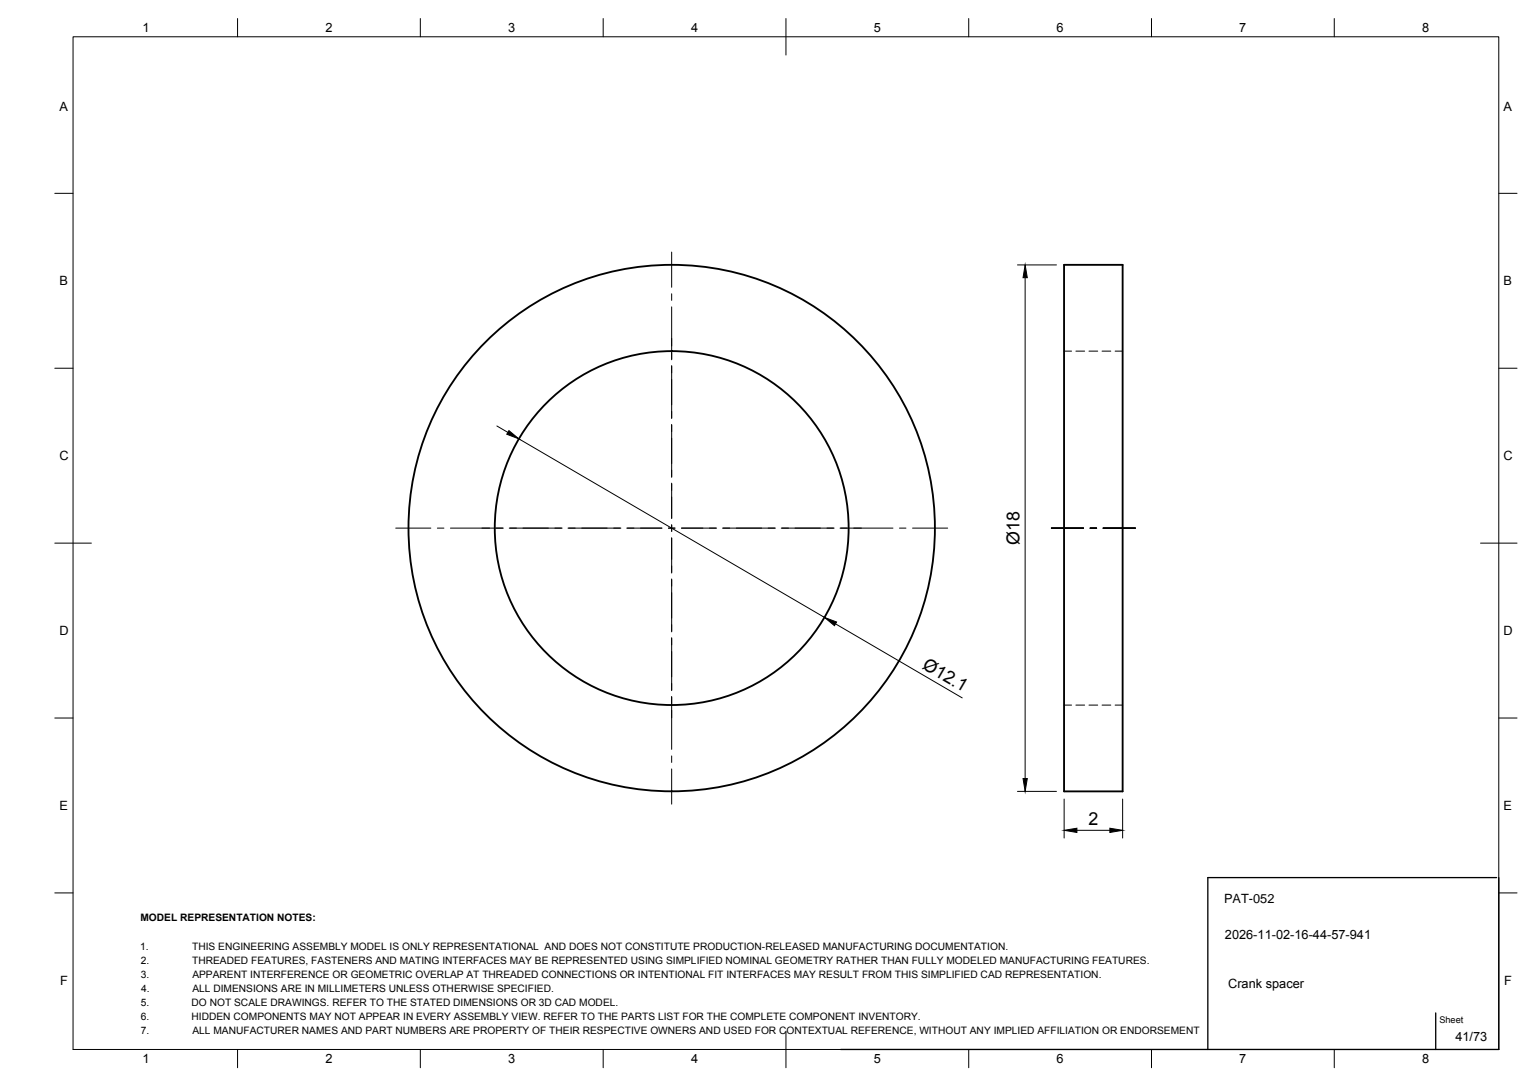
ISO-10303-21;
HEADER;
/* Generated by software containing ST-Developer
 * from STEP Tools, Inc. (www.steptools.com) 
 */

FILE_DESCRIPTION(
/* description */ ('Hand-crank gear train demonstrator'),
/* implementation_level */ '2;1');

FILE_NAME(
/* name */ 'Crank spacer.step',
/* time_stamp */ '2026-10-28T03:22:13-07:00',
/* author */ (''),
/* organization */ (''),
/* preprocessor_version */ 'ST-DEVELOPER v20.2',
/* originating_system */ 'Autodesk Translation Framework v15.17.0.0',
/* authorisation */ '');

FILE_SCHEMA (('AUTOMOTIVE_DESIGN { 1 0 10303 214 3 1 1 }'));
ENDSEC;

DATA;
#10=MECHANICAL_DESIGN_GEOMETRIC_PRESENTATION_REPRESENTATION('',(#1237),#62758);
#1094=SHAPE_REPRESENTATION_RELATIONSHIP('SRR','None',#63069,#1158);
#1158=ADVANCED_BREP_SHAPE_REPRESENTATION('',(#1313),#62723);
#1237=STYLED_ITEM('',(#63455),#1313);
#1313=MANIFOLD_SOLID_BREP('Body1',#16420);
#1560=FACE_BOUND('',#3751,.T.);
#1561=FACE_BOUND('',#3753,.T.);
#1915=PLANE('',#18069);
#1916=PLANE('',#18070);
#2594=FACE_OUTER_BOUND('',#3748,.T.);
#2595=FACE_OUTER_BOUND('',#3749,.T.);
#2596=FACE_OUTER_BOUND('',#3750,.T.);
#2597=FACE_OUTER_BOUND('',#3752,.T.);
#3748=EDGE_LOOP('',(#12897,#12898,#12899,#12900));
#3749=EDGE_LOOP('',(#12901,#12902,#12903,#12904));
#3750=EDGE_LOOP('',(#12905));
#3751=EDGE_LOOP('',(#12906));
#3752=EDGE_LOOP('',(#12907));
#3753=EDGE_LOOP('',(#12908));
#4896=LINE('',#26250,#6028);
#4897=LINE('',#26256,#6029);
#6028=VECTOR('',#21255,0.605);
#6029=VECTOR('',#21262,0.9);
#6935=CIRCLE('',#18064,0.605);
#6936=CIRCLE('',#18065,0.605);
#6937=CIRCLE('',#18067,0.9);
#6938=CIRCLE('',#18068,0.9);
#7914=VERTEX_POINT('',#26247);
#7915=VERTEX_POINT('',#26249);
#7916=VERTEX_POINT('',#26253);
#7917=VERTEX_POINT('',#26255);
#9700=EDGE_CURVE('',#7914,#7914,#6935,.T.);
#9701=EDGE_CURVE('',#7914,#7915,#4896,.T.);
#9702=EDGE_CURVE('',#7915,#7915,#6936,.T.);
#9703=EDGE_CURVE('',#7916,#7916,#6937,.T.);
#9704=EDGE_CURVE('',#7916,#7917,#4897,.T.);
#9705=EDGE_CURVE('',#7917,#7917,#6938,.T.);
#12897=ORIENTED_EDGE('',*,*,#9700,.F.);
#12898=ORIENTED_EDGE('',*,*,#9701,.T.);
#12899=ORIENTED_EDGE('',*,*,#9702,.T.);
#12900=ORIENTED_EDGE('',*,*,#9701,.F.);
#12901=ORIENTED_EDGE('',*,*,#9703,.F.);
#12902=ORIENTED_EDGE('',*,*,#9704,.T.);
#12903=ORIENTED_EDGE('',*,*,#9705,.T.);
#12904=ORIENTED_EDGE('',*,*,#9704,.F.);
#12905=ORIENTED_EDGE('',*,*,#9703,.T.);
#12906=ORIENTED_EDGE('',*,*,#9700,.T.);
#12907=ORIENTED_EDGE('',*,*,#9705,.F.);
#12908=ORIENTED_EDGE('',*,*,#9702,.F.);
#15305=CYLINDRICAL_SURFACE('',#18063,0.605);
#15306=CYLINDRICAL_SURFACE('',#18066,0.9);
#15904=ADVANCED_FACE('',(#2594),#15305,.F.);
#15905=ADVANCED_FACE('',(#2595),#15306,.T.);
#15906=ADVANCED_FACE('',(#2596,#1560),#1915,.T.);
#15907=ADVANCED_FACE('',(#2597,#1561),#1916,.F.);
#16420=CLOSED_SHELL('',(#15904,#15905,#15906,#15907));
#18062=AXIS2_PLACEMENT_3D('',#26245,#21249,#21250);
#18063=AXIS2_PLACEMENT_3D('',#26246,#21251,#21252);
#18064=AXIS2_PLACEMENT_3D('',#26248,#21253,#21254);
#18065=AXIS2_PLACEMENT_3D('',#26251,#21256,#21257);
#18066=AXIS2_PLACEMENT_3D('',#26252,#21258,#21259);
#18067=AXIS2_PLACEMENT_3D('',#26254,#21260,#21261);
#18068=AXIS2_PLACEMENT_3D('',#26257,#21263,#21264);
#18069=AXIS2_PLACEMENT_3D('',#26258,#21265,#21266);
#18070=AXIS2_PLACEMENT_3D('',#26259,#21267,#21268);
#21249=DIRECTION('axis',(0.,0.,1.));
#21250=DIRECTION('refdir',(1.,0.,0.));
#21251=DIRECTION('center_axis',(0.,1.,0.));
#21252=DIRECTION('ref_axis',(1.,0.,0.));
#21253=DIRECTION('center_axis',(0.,-1.,0.));
#21254=DIRECTION('ref_axis',(1.,0.,0.));
#21255=DIRECTION('',(0.,-1.,0.));
#21256=DIRECTION('center_axis',(0.,-1.,0.));
#21257=DIRECTION('ref_axis',(1.,0.,0.));
#21258=DIRECTION('center_axis',(0.,1.,0.));
#21259=DIRECTION('ref_axis',(1.,0.,0.));
#21260=DIRECTION('center_axis',(0.,1.,0.));
#21261=DIRECTION('ref_axis',(1.,0.,0.));
#21262=DIRECTION('',(0.,-1.,0.));
#21263=DIRECTION('center_axis',(0.,1.,0.));
#21264=DIRECTION('ref_axis',(1.,0.,0.));
#21265=DIRECTION('center_axis',(0.,1.,0.));
#21266=DIRECTION('ref_axis',(1.,0.,0.));
#21267=DIRECTION('center_axis',(0.,1.,0.));
#21268=DIRECTION('ref_axis',(1.,0.,0.));
#26245=CARTESIAN_POINT('',(0.,0.,0.));
#26246=CARTESIAN_POINT('Origin',(0.,3.2,9.));
#26247=CARTESIAN_POINT('',(-0.605,3.4,9.));
#26248=CARTESIAN_POINT('Origin',(0.,3.4,9.));
#26249=CARTESIAN_POINT('',(-0.605,3.2,9.));
#26250=CARTESIAN_POINT('',(-0.605,3.2,9.));
#26251=CARTESIAN_POINT('Origin',(0.,3.2,9.));
#26252=CARTESIAN_POINT('Origin',(0.,3.2,9.));
#26253=CARTESIAN_POINT('',(-0.9,3.4,9.));
#26254=CARTESIAN_POINT('Origin',(0.,3.4,9.));
#26255=CARTESIAN_POINT('',(-0.9,3.2,9.));
#26256=CARTESIAN_POINT('',(-0.9,3.2,9.));
#26257=CARTESIAN_POINT('Origin',(0.,3.2,9.));
#26258=CARTESIAN_POINT('Origin',(0.,3.4,9.));
#26259=CARTESIAN_POINT('Origin',(0.,3.2,9.));
#62649=UNCERTAINTY_MEASURE_WITH_UNIT(LENGTH_MEASURE(0.001),#62759,
'DISTANCE_ACCURACY_VALUE',
'Maximum model space distance between geometric entities at asserted c
onnectivities');
#62684=UNCERTAINTY_MEASURE_WITH_UNIT(LENGTH_MEASURE(0.001),#62759,
'DISTANCE_ACCURACY_VALUE',
'Maximum model space distance between geometric entities at asserted c
onnectivities');
#62723=(
GEOMETRIC_REPRESENTATION_CONTEXT(3)
GLOBAL_UNCERTAINTY_ASSIGNED_CONTEXT((#62649))
GLOBAL_UNIT_ASSIGNED_CONTEXT((#62759,#62761,#62762))
REPRESENTATION_CONTEXT('','3D')
);
#62758=(
GEOMETRIC_REPRESENTATION_CONTEXT(3)
GLOBAL_UNCERTAINTY_ASSIGNED_CONTEXT((#62684))
GLOBAL_UNIT_ASSIGNED_CONTEXT((#62759,#62761,#62762))
REPRESENTATION_CONTEXT('','3D')
);
#62759=(
LENGTH_UNIT()
NAMED_UNIT(*)
SI_UNIT(.CENTI.,.METRE.)
);
#62761=(
NAMED_UNIT(*)
PLANE_ANGLE_UNIT()
SI_UNIT($,.RADIAN.)
);
#62762=(
NAMED_UNIT(*)
SI_UNIT($,.STERADIAN.)
SOLID_ANGLE_UNIT()
);
#62801=SHAPE_DEFINITION_REPRESENTATION(#62884,#63069);
#62884=PRODUCT_DEFINITION_SHAPE('',$,#63143);
#63069=SHAPE_REPRESENTATION('',(#18062),#62723);
#63104=PRODUCT_DEFINITION_CONTEXT('part definition',#63325,'design');
#63143=PRODUCT_DEFINITION('Crank spacer','Crank spacer',#63216,#63104);
#63216=PRODUCT_DEFINITION_FORMATION('',$,#63365);
#63325=APPLICATION_CONTEXT(
'Core Data for Automotive Mechanical Design Process');
#63326=PRODUCT_CONTEXT('part definition',#63325,'mechanical');
#63365=PRODUCT('Crank spacer','Crank spacer','Crank spacer',(#63326));
#63449=COLOUR_RGB('Sky Blue',0.24,0.69,0.87);
#63450=FILL_AREA_STYLE_COLOUR('',#63449);
#63451=FILL_AREA_STYLE('',(#63450));
#63452=SURFACE_STYLE_FILL_AREA(#63451);
#63453=SURFACE_SIDE_STYLE('',(#63452));
#63454=SURFACE_STYLE_USAGE(.BOTH.,#63453);
#63455=PRESENTATION_STYLE_ASSIGNMENT((#63454));
ENDSEC;
END-ISO-10303-21;
